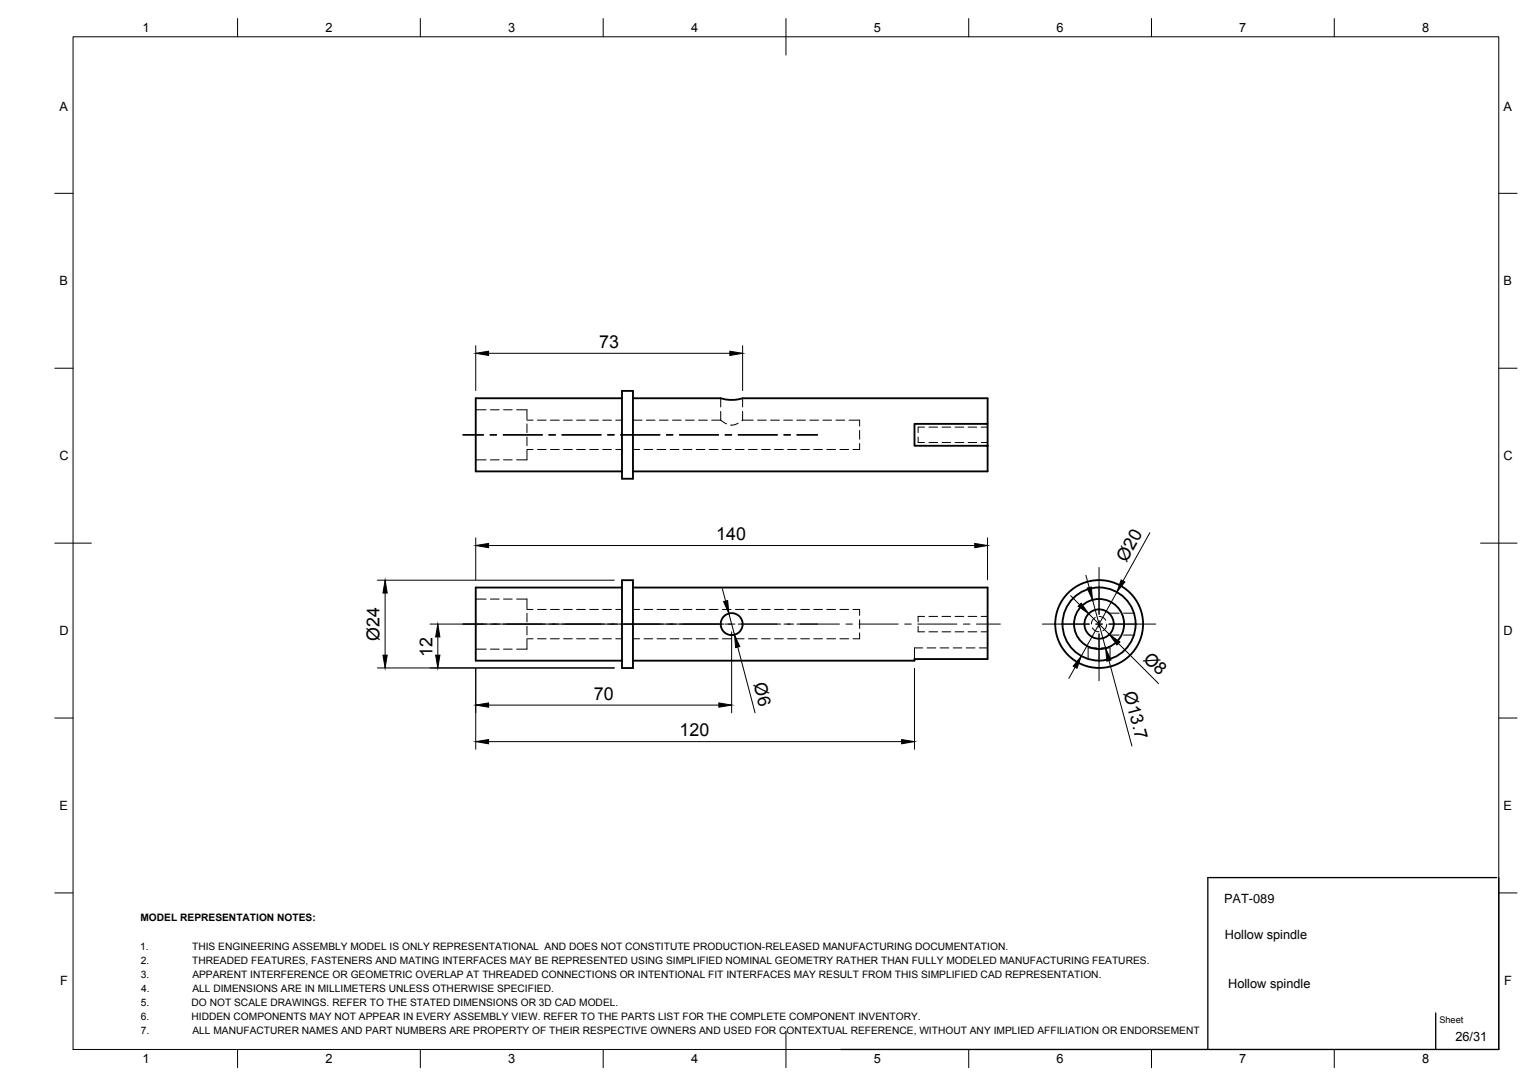
ISO-10303-21;
HEADER;
/* Generated by software containing ST-Developer
 * from STEP Tools, Inc. (www.steptools.com) 
 */

FILE_DESCRIPTION(
/* description */ ('Rotary union on bearing shaft'),
/* implementation_level */ '2;1');

FILE_NAME(
/* name */ 'Hollow spindle.step',
/* time_stamp */ '2026-10-28T03:24:01-07:00',
/* author */ (''),
/* organization */ (''),
/* preprocessor_version */ 'ST-DEVELOPER v20.2',
/* originating_system */ 'Autodesk Translation Framework v15.17.0.0',
/* authorisation */ '');

FILE_SCHEMA (('AUTOMOTIVE_DESIGN { 1 0 10303 214 3 1 1 }'));
ENDSEC;

DATA;
#10=MECHANICAL_DESIGN_GEOMETRIC_PRESENTATION_REPRESENTATION('',(#339),#9448);
#251=B_SPLINE_CURVE_WITH_KNOTS('',3,(#8795,#8796,#8797,#8798,#8799,#8800,
#8801,#8802,#8803,#8804,#8805,#8806,#8807,#8808,#8809,#8810,#8811,#8812),
 .UNSPECIFIED.,.F.,.F.,(4,2,2,2,2,2,2,2,4),(0.,0.113783176196775,0.22756635239355,
0.34131563198115,0.455064911568751,0.568814191156351,0.682563470743952,
0.796346646940726,0.910129823137501),.UNSPECIFIED.);
#252=B_SPLINE_CURVE_WITH_KNOTS('',3,(#8813,#8814,#8815,#8816,#8817,#8818,
#8819,#8820,#8821,#8822,#8823,#8824,#8825,#8826,#8827,#8828,#8829,#8830),
 .UNSPECIFIED.,.F.,.F.,(4,2,2,2,2,2,2,2,4),(0.910129823137501,1.02391299933428,
1.13769617553105,1.25144545511865,1.36519473470625,1.47894401429385,1.59269329388145,
1.70647647007823,1.820259646275),.UNSPECIFIED.);
#253=B_SPLINE_CURVE_WITH_KNOTS('',3,(#8865,#8866,#8867,#8868,#8869,#8870,
#8871,#8872,#8873,#8874,#8875,#8876,#8877,#8878,#8879,#8880,#8881,#8882,
#8883,#8884,#8885,#8886),.UNSPECIFIED.,.F.,.F.,(4,2,2,2,2,2,2,2,2,2,4),
(0.,0.0604340316452086,0.120868063290417,0.241736126580834,0.36006196705804,
0.478387807535245,0.596713648012451,0.715039488489656,0.835907551780074,
0.896341583425282,0.956775615070491),.UNSPECIFIED.);
#254=B_SPLINE_CURVE_WITH_KNOTS('',3,(#8887,#8888,#8889,#8890,#8891,#8892,
#8893,#8894,#8895,#8896,#8897,#8898,#8899,#8900,#8901,#8902,#8903,#8904,
#8905,#8906,#8907,#8908),.UNSPECIFIED.,.F.,.F.,(4,2,2,2,2,2,2,2,2,2,4),
(0.956775615070491,1.0172096467157,1.07764367836091,1.19851174165133,1.31683758212853,
1.43516342260574,1.55348926308294,1.67181510356015,1.79268316685056,1.85311719849577,
1.91355123014098),.UNSPECIFIED.);
#277=SHAPE_REPRESENTATION_RELATIONSHIP('SRR','None',#9579,#304);
#304=ADVANCED_BREP_SHAPE_REPRESENTATION('',(#372),#9439);
#339=STYLED_ITEM('',(#9764),#372);
#372=MANIFOLD_SOLID_BREP('Body1',#4896);
#455=FACE_BOUND('',#1233,.T.);
#456=FACE_BOUND('',#1235,.T.);
#457=FACE_BOUND('',#1238,.T.);
#458=FACE_BOUND('',#1245,.T.);
#459=FACE_BOUND('',#1248,.T.);
#460=FACE_BOUND('',#1251,.T.);
#461=FACE_BOUND('',#1253,.T.);
#589=PLANE('',#5618);
#590=PLANE('',#5619);
#591=PLANE('',#5620);
#592=PLANE('',#5622);
#593=PLANE('',#5623);
#594=PLANE('',#5628);
#595=PLANE('',#5630);
#596=PLANE('',#5632);
#597=PLANE('',#5635);
#598=PLANE('',#5645);
#599=PLANE('',#5649);
#600=PLANE('',#5650);
#601=PLANE('',#5651);
#852=FACE_OUTER_BOUND('',#1226,.T.);
#853=FACE_OUTER_BOUND('',#1227,.T.);
#854=FACE_OUTER_BOUND('',#1228,.T.);
#855=FACE_OUTER_BOUND('',#1229,.T.);
#856=FACE_OUTER_BOUND('',#1230,.T.);
#857=FACE_OUTER_BOUND('',#1231,.T.);
#858=FACE_OUTER_BOUND('',#1232,.T.);
#859=FACE_OUTER_BOUND('',#1234,.T.);
#860=FACE_OUTER_BOUND('',#1236,.T.);
#861=FACE_OUTER_BOUND('',#1237,.T.);
#862=FACE_OUTER_BOUND('',#1239,.T.);
#863=FACE_OUTER_BOUND('',#1240,.T.);
#864=FACE_OUTER_BOUND('',#1241,.T.);
#865=FACE_OUTER_BOUND('',#1242,.T.);
#866=FACE_OUTER_BOUND('',#1243,.T.);
#867=FACE_OUTER_BOUND('',#1244,.T.);
#868=FACE_OUTER_BOUND('',#1246,.T.);
#869=FACE_OUTER_BOUND('',#1247,.T.);
#870=FACE_OUTER_BOUND('',#1249,.T.);
#871=FACE_OUTER_BOUND('',#1250,.T.);
#872=FACE_OUTER_BOUND('',#1252,.T.);
#1226=EDGE_LOOP('',(#4063,#4064,#4065,#4066));
#1227=EDGE_LOOP('',(#4067));
#1228=EDGE_LOOP('',(#4068,#4069,#4070,#4071));
#1229=EDGE_LOOP('',(#4072,#4073,#4074,#4075));
#1230=EDGE_LOOP('',(#4076,#4077,#4078,#4079));
#1231=EDGE_LOOP('',(#4080,#4081,#4082,#4083));
#1232=EDGE_LOOP('',(#4084,#4085,#4086,#4087,#4088,#4089,#4090,#4091));
#1233=EDGE_LOOP('',(#4092,#4093));
#1234=EDGE_LOOP('',(#4094));
#1235=EDGE_LOOP('',(#4095));
#1236=EDGE_LOOP('',(#4096));
#1237=EDGE_LOOP('',(#4097));
#1238=EDGE_LOOP('',(#4098));
#1239=EDGE_LOOP('',(#4099));
#1240=EDGE_LOOP('',(#4100,#4101,#4102,#4103));
#1241=EDGE_LOOP('',(#4104,#4105,#4106,#4107));
#1242=EDGE_LOOP('',(#4108,#4109,#4110,#4111));
#1243=EDGE_LOOP('',(#4112,#4113,#4114,#4115));
#1244=EDGE_LOOP('',(#4116));
#1245=EDGE_LOOP('',(#4117));
#1246=EDGE_LOOP('',(#4118,#4119,#4120,#4121,#4122,#4123));
#1247=EDGE_LOOP('',(#4124,#4125,#4126,#4127));
#1248=EDGE_LOOP('',(#4128,#4129));
#1249=EDGE_LOOP('',(#4130));
#1250=EDGE_LOOP('',(#4131,#4132,#4133,#4134,#4135));
#1251=EDGE_LOOP('',(#4136));
#1252=EDGE_LOOP('',(#4137));
#1253=EDGE_LOOP('',(#4138));
#1546=LINE('',#8760,#1866);
#1547=LINE('',#8766,#1867);
#1548=LINE('',#8768,#1868);
#1549=LINE('',#8770,#1869);
#1550=LINE('',#8771,#1870);
#1551=LINE('',#8776,#1871);
#1552=LINE('',#8777,#1872);
#1553=LINE('',#8780,#1873);
#1554=LINE('',#8782,#1874);
#1555=LINE('',#8783,#1875);
#1556=LINE('',#8785,#1876);
#1557=LINE('',#8790,#1877);
#1558=LINE('',#8846,#1878);
#1559=LINE('',#8850,#1879);
#1560=LINE('',#8853,#1880);
#1561=LINE('',#8859,#1881);
#1562=LINE('',#8909,#1882);
#1563=LINE('',#8912,#1883);
#1866=VECTOR('',#6839,0.21);
#1867=VECTOR('',#6846,1.);
#1868=VECTOR('',#6847,1.);
#1869=VECTOR('',#6848,1.);
#1870=VECTOR('',#6849,1.);
#1871=VECTOR('',#6854,1.);
#1872=VECTOR('',#6855,1.);
#1873=VECTOR('',#6858,1.);
#1874=VECTOR('',#6859,1.);
#1875=VECTOR('',#6860,1.);
#1876=VECTOR('',#6863,1.);
#1877=VECTOR('',#6868,1.);
#1878=VECTOR('',#6893,1.2);
#1879=VECTOR('',#6898,0.4);
#1880=VECTOR('',#6901,1.);
#1881=VECTOR('',#6908,0.685);
#1882=VECTOR('',#6915,0.3);
#1883=VECTOR('',#6918,0.4);
#2188=CIRCLE('',#5616,0.21);
#2189=CIRCLE('',#5617,0.21);
#2190=CIRCLE('',#5621,1.);
#2191=CIRCLE('',#5625,1.);
#2192=CIRCLE('',#5626,1.);
#2193=CIRCLE('',#5627,1.);
#2194=CIRCLE('',#5629,1.2);
#2195=CIRCLE('',#5631,0.4);
#2196=CIRCLE('',#5633,1.2);
#2197=CIRCLE('',#5634,1.);
#2198=CIRCLE('',#5636,0.4);
#2199=CIRCLE('',#5639,0.4);
#2200=CIRCLE('',#5641,1.);
#2201=CIRCLE('',#5643,0.685);
#2202=CIRCLE('',#5644,0.685);
#2203=CIRCLE('',#5648,0.4);
#2524=VERTEX_POINT('',#8757);
#2525=VERTEX_POINT('',#8759);
#2526=VERTEX_POINT('',#8764);
#2527=VERTEX_POINT('',#8765);
#2528=VERTEX_POINT('',#8767);
#2529=VERTEX_POINT('',#8769);
#2530=VERTEX_POINT('',#8773);
#2531=VERTEX_POINT('',#8775);
#2532=VERTEX_POINT('',#8779);
#2533=VERTEX_POINT('',#8781);
#2534=VERTEX_POINT('',#8787);
#2535=VERTEX_POINT('',#8789);
#2536=VERTEX_POINT('',#8793);
#2537=VERTEX_POINT('',#8794);
#2538=VERTEX_POINT('',#8832);
#2539=VERTEX_POINT('',#8835);
#2540=VERTEX_POINT('',#8838);
#2541=VERTEX_POINT('',#8840);
#2542=VERTEX_POINT('',#8843);
#2543=VERTEX_POINT('',#8848);
#2544=VERTEX_POINT('',#8852);
#2545=VERTEX_POINT('',#8856);
#2546=VERTEX_POINT('',#8858);
#2547=VERTEX_POINT('',#8863);
#2548=VERTEX_POINT('',#8864);
#2549=VERTEX_POINT('',#8911);
#3059=EDGE_CURVE('',#2524,#2524,#2188,.T.);
#3060=EDGE_CURVE('',#2524,#2525,#1546,.T.);
#3061=EDGE_CURVE('',#2525,#2525,#2189,.T.);
#3062=EDGE_CURVE('',#2526,#2527,#1547,.T.);
#3063=EDGE_CURVE('',#2528,#2526,#1548,.T.);
#3064=EDGE_CURVE('',#2529,#2528,#1549,.T.);
#3065=EDGE_CURVE('',#2529,#2527,#1550,.T.);
#3066=EDGE_CURVE('',#2527,#2530,#2190,.T.);
#3067=EDGE_CURVE('',#2531,#2529,#1551,.T.);
#3068=EDGE_CURVE('',#2530,#2531,#1552,.T.);
#3069=EDGE_CURVE('',#2530,#2532,#1553,.T.);
#3070=EDGE_CURVE('',#2531,#2533,#1554,.T.);
#3071=EDGE_CURVE('',#2532,#2533,#1555,.T.);
#3072=EDGE_CURVE('',#2533,#2528,#1556,.T.);
#3073=EDGE_CURVE('',#2534,#2532,#2191,.T.);
#3074=EDGE_CURVE('',#2534,#2535,#1557,.T.);
#3075=EDGE_CURVE('',#2535,#2535,#2192,.T.);
#3076=EDGE_CURVE('',#2526,#2534,#2193,.T.);
#3077=EDGE_CURVE('',#2536,#2537,#251,.T.);
#3078=EDGE_CURVE('',#2537,#2536,#252,.T.);
#3079=EDGE_CURVE('',#2538,#2538,#2194,.T.);
#3080=EDGE_CURVE('',#2539,#2539,#2195,.T.);
#3081=EDGE_CURVE('',#2540,#2540,#2196,.T.);
#3082=EDGE_CURVE('',#2541,#2541,#2197,.T.);
#3083=EDGE_CURVE('',#2542,#2542,#2198,.T.);
#3084=EDGE_CURVE('',#2538,#2540,#1558,.T.);
#3085=EDGE_CURVE('',#2543,#2543,#2199,.T.);
#3086=EDGE_CURVE('',#2543,#2542,#1559,.T.);
#3087=EDGE_CURVE('',#2541,#2544,#1560,.T.);
#3088=EDGE_CURVE('',#2544,#2544,#2200,.T.);
#3089=EDGE_CURVE('',#2545,#2545,#2201,.T.);
#3090=EDGE_CURVE('',#2545,#2546,#1561,.T.);
#3091=EDGE_CURVE('',#2546,#2546,#2202,.T.);
#3092=EDGE_CURVE('',#2547,#2548,#253,.T.);
#3093=EDGE_CURVE('',#2548,#2547,#254,.T.);
#3094=EDGE_CURVE('',#2548,#2537,#1562,.T.);
#3095=EDGE_CURVE('',#2539,#2549,#1563,.T.);
#3096=EDGE_CURVE('',#2549,#2549,#2203,.T.);
#4063=ORIENTED_EDGE('',*,*,#3059,.F.);
#4064=ORIENTED_EDGE('',*,*,#3060,.T.);
#4065=ORIENTED_EDGE('',*,*,#3061,.F.);
#4066=ORIENTED_EDGE('',*,*,#3060,.F.);
#4067=ORIENTED_EDGE('',*,*,#3059,.T.);
#4068=ORIENTED_EDGE('',*,*,#3062,.F.);
#4069=ORIENTED_EDGE('',*,*,#3063,.F.);
#4070=ORIENTED_EDGE('',*,*,#3064,.F.);
#4071=ORIENTED_EDGE('',*,*,#3065,.T.);
#4072=ORIENTED_EDGE('',*,*,#3066,.F.);
#4073=ORIENTED_EDGE('',*,*,#3065,.F.);
#4074=ORIENTED_EDGE('',*,*,#3067,.F.);
#4075=ORIENTED_EDGE('',*,*,#3068,.F.);
#4076=ORIENTED_EDGE('',*,*,#3069,.F.);
#4077=ORIENTED_EDGE('',*,*,#3068,.T.);
#4078=ORIENTED_EDGE('',*,*,#3070,.T.);
#4079=ORIENTED_EDGE('',*,*,#3071,.F.);
#4080=ORIENTED_EDGE('',*,*,#3067,.T.);
#4081=ORIENTED_EDGE('',*,*,#3064,.T.);
#4082=ORIENTED_EDGE('',*,*,#3072,.F.);
#4083=ORIENTED_EDGE('',*,*,#3070,.F.);
#4084=ORIENTED_EDGE('',*,*,#3062,.T.);
#4085=ORIENTED_EDGE('',*,*,#3066,.T.);
#4086=ORIENTED_EDGE('',*,*,#3069,.T.);
#4087=ORIENTED_EDGE('',*,*,#3073,.F.);
#4088=ORIENTED_EDGE('',*,*,#3074,.T.);
#4089=ORIENTED_EDGE('',*,*,#3075,.T.);
#4090=ORIENTED_EDGE('',*,*,#3074,.F.);
#4091=ORIENTED_EDGE('',*,*,#3076,.F.);
#4092=ORIENTED_EDGE('',*,*,#3077,.T.);
#4093=ORIENTED_EDGE('',*,*,#3078,.T.);
#4094=ORIENTED_EDGE('',*,*,#3079,.T.);
#4095=ORIENTED_EDGE('',*,*,#3075,.F.);
#4096=ORIENTED_EDGE('',*,*,#3080,.F.);
#4097=ORIENTED_EDGE('',*,*,#3081,.F.);
#4098=ORIENTED_EDGE('',*,*,#3082,.F.);
#4099=ORIENTED_EDGE('',*,*,#3083,.F.);
#4100=ORIENTED_EDGE('',*,*,#3079,.F.);
#4101=ORIENTED_EDGE('',*,*,#3084,.T.);
#4102=ORIENTED_EDGE('',*,*,#3081,.T.);
#4103=ORIENTED_EDGE('',*,*,#3084,.F.);
#4104=ORIENTED_EDGE('',*,*,#3085,.T.);
#4105=ORIENTED_EDGE('',*,*,#3086,.T.);
#4106=ORIENTED_EDGE('',*,*,#3083,.T.);
#4107=ORIENTED_EDGE('',*,*,#3086,.F.);
#4108=ORIENTED_EDGE('',*,*,#3082,.T.);
#4109=ORIENTED_EDGE('',*,*,#3087,.T.);
#4110=ORIENTED_EDGE('',*,*,#3088,.T.);
#4111=ORIENTED_EDGE('',*,*,#3087,.F.);
#4112=ORIENTED_EDGE('',*,*,#3089,.F.);
#4113=ORIENTED_EDGE('',*,*,#3090,.T.);
#4114=ORIENTED_EDGE('',*,*,#3091,.T.);
#4115=ORIENTED_EDGE('',*,*,#3090,.F.);
#4116=ORIENTED_EDGE('',*,*,#3091,.F.);
#4117=ORIENTED_EDGE('',*,*,#3085,.F.);
#4118=ORIENTED_EDGE('',*,*,#3092,.F.);
#4119=ORIENTED_EDGE('',*,*,#3093,.F.);
#4120=ORIENTED_EDGE('',*,*,#3094,.T.);
#4121=ORIENTED_EDGE('',*,*,#3077,.F.);
#4122=ORIENTED_EDGE('',*,*,#3078,.F.);
#4123=ORIENTED_EDGE('',*,*,#3094,.F.);
#4124=ORIENTED_EDGE('',*,*,#3080,.T.);
#4125=ORIENTED_EDGE('',*,*,#3095,.T.);
#4126=ORIENTED_EDGE('',*,*,#3096,.T.);
#4127=ORIENTED_EDGE('',*,*,#3095,.F.);
#4128=ORIENTED_EDGE('',*,*,#3092,.T.);
#4129=ORIENTED_EDGE('',*,*,#3093,.T.);
#4130=ORIENTED_EDGE('',*,*,#3096,.F.);
#4131=ORIENTED_EDGE('',*,*,#3063,.T.);
#4132=ORIENTED_EDGE('',*,*,#3076,.T.);
#4133=ORIENTED_EDGE('',*,*,#3073,.T.);
#4134=ORIENTED_EDGE('',*,*,#3071,.T.);
#4135=ORIENTED_EDGE('',*,*,#3072,.T.);
#4136=ORIENTED_EDGE('',*,*,#3061,.T.);
#4137=ORIENTED_EDGE('',*,*,#3088,.F.);
#4138=ORIENTED_EDGE('',*,*,#3089,.T.);
#4541=CYLINDRICAL_SURFACE('',#5615,0.21);
#4542=CYLINDRICAL_SURFACE('',#5624,1.);
#4543=CYLINDRICAL_SURFACE('',#5637,1.2);
#4544=CYLINDRICAL_SURFACE('',#5638,0.4);
#4545=CYLINDRICAL_SURFACE('',#5640,1.);
#4546=CYLINDRICAL_SURFACE('',#5642,0.685);
#4547=CYLINDRICAL_SURFACE('',#5646,0.3);
#4548=CYLINDRICAL_SURFACE('',#5647,0.4);
#4765=ADVANCED_FACE('',(#852),#4541,.F.);
#4766=ADVANCED_FACE('',(#853),#589,.T.);
#4767=ADVANCED_FACE('',(#854),#590,.F.);
#4768=ADVANCED_FACE('',(#855),#591,.T.);
#4769=ADVANCED_FACE('',(#856),#592,.F.);
#4770=ADVANCED_FACE('',(#857),#593,.F.);
#4771=ADVANCED_FACE('',(#858,#455),#4542,.T.);
#4772=ADVANCED_FACE('',(#859,#456),#594,.T.);
#4773=ADVANCED_FACE('',(#860),#595,.T.);
#4774=ADVANCED_FACE('',(#861,#457),#596,.F.);
#4775=ADVANCED_FACE('',(#862),#597,.F.);
#4776=ADVANCED_FACE('',(#863),#4543,.T.);
#4777=ADVANCED_FACE('',(#864),#4544,.F.);
#4778=ADVANCED_FACE('',(#865),#4545,.T.);
#4779=ADVANCED_FACE('',(#866),#4546,.F.);
#4780=ADVANCED_FACE('',(#867,#458),#598,.F.);
#4781=ADVANCED_FACE('',(#868),#4547,.F.);
#4782=ADVANCED_FACE('',(#869,#459),#4548,.F.);
#4783=ADVANCED_FACE('',(#870),#599,.F.);
#4784=ADVANCED_FACE('',(#871,#460),#600,.T.);
#4785=ADVANCED_FACE('',(#872,#461),#601,.F.);
#4896=CLOSED_SHELL('',(#4765,#4766,#4767,#4768,#4769,#4770,#4771,#4772,
#4773,#4774,#4775,#4776,#4777,#4778,#4779,#4780,#4781,#4782,#4783,#4784,
#4785));
#5614=AXIS2_PLACEMENT_3D('',#8755,#6833,#6834);
#5615=AXIS2_PLACEMENT_3D('',#8756,#6835,#6836);
#5616=AXIS2_PLACEMENT_3D('',#8758,#6837,#6838);
#5617=AXIS2_PLACEMENT_3D('',#8761,#6840,#6841);
#5618=AXIS2_PLACEMENT_3D('',#8762,#6842,#6843);
#5619=AXIS2_PLACEMENT_3D('',#8763,#6844,#6845);
#5620=AXIS2_PLACEMENT_3D('',#8772,#6850,#6851);
#5621=AXIS2_PLACEMENT_3D('',#8774,#6852,#6853);
#5622=AXIS2_PLACEMENT_3D('',#8778,#6856,#6857);
#5623=AXIS2_PLACEMENT_3D('',#8784,#6861,#6862);
#5624=AXIS2_PLACEMENT_3D('',#8786,#6864,#6865);
#5625=AXIS2_PLACEMENT_3D('',#8788,#6866,#6867);
#5626=AXIS2_PLACEMENT_3D('',#8791,#6869,#6870);
#5627=AXIS2_PLACEMENT_3D('',#8792,#6871,#6872);
#5628=AXIS2_PLACEMENT_3D('',#8831,#6873,#6874);
#5629=AXIS2_PLACEMENT_3D('',#8833,#6875,#6876);
#5630=AXIS2_PLACEMENT_3D('',#8834,#6877,#6878);
#5631=AXIS2_PLACEMENT_3D('',#8836,#6879,#6880);
#5632=AXIS2_PLACEMENT_3D('',#8837,#6881,#6882);
#5633=AXIS2_PLACEMENT_3D('',#8839,#6883,#6884);
#5634=AXIS2_PLACEMENT_3D('',#8841,#6885,#6886);
#5635=AXIS2_PLACEMENT_3D('',#8842,#6887,#6888);
#5636=AXIS2_PLACEMENT_3D('',#8844,#6889,#6890);
#5637=AXIS2_PLACEMENT_3D('',#8845,#6891,#6892);
#5638=AXIS2_PLACEMENT_3D('',#8847,#6894,#6895);
#5639=AXIS2_PLACEMENT_3D('',#8849,#6896,#6897);
#5640=AXIS2_PLACEMENT_3D('',#8851,#6899,#6900);
#5641=AXIS2_PLACEMENT_3D('',#8854,#6902,#6903);
#5642=AXIS2_PLACEMENT_3D('',#8855,#6904,#6905);
#5643=AXIS2_PLACEMENT_3D('',#8857,#6906,#6907);
#5644=AXIS2_PLACEMENT_3D('',#8860,#6909,#6910);
#5645=AXIS2_PLACEMENT_3D('',#8861,#6911,#6912);
#5646=AXIS2_PLACEMENT_3D('',#8862,#6913,#6914);
#5647=AXIS2_PLACEMENT_3D('',#8910,#6916,#6917);
#5648=AXIS2_PLACEMENT_3D('',#8913,#6919,#6920);
#5649=AXIS2_PLACEMENT_3D('',#8914,#6921,#6922);
#5650=AXIS2_PLACEMENT_3D('',#8915,#6923,#6924);
#5651=AXIS2_PLACEMENT_3D('',#8916,#6925,#6926);
#6833=DIRECTION('axis',(0.,0.,1.));
#6834=DIRECTION('refdir',(1.,0.,0.));
#6835=DIRECTION('center_axis',(0.,1.,0.));
#6836=DIRECTION('ref_axis',(1.,0.,0.));
#6837=DIRECTION('center_axis',(0.,1.,0.));
#6838=DIRECTION('ref_axis',(1.,0.,0.));
#6839=DIRECTION('',(0.,1.,0.));
#6840=DIRECTION('center_axis',(0.,-1.,0.));
#6841=DIRECTION('ref_axis',(1.,0.,0.));
#6842=DIRECTION('center_axis',(0.,1.,0.));
#6843=DIRECTION('ref_axis',(1.,0.,0.));
#6844=DIRECTION('center_axis',(-1.,0.,0.));
#6845=DIRECTION('ref_axis',(0.,0.,1.));
#6846=DIRECTION('',(0.,-1.,0.));
#6847=DIRECTION('',(0.,0.,-1.));
#6848=DIRECTION('',(0.,1.,0.));
#6849=DIRECTION('',(0.,0.,-1.));
#6850=DIRECTION('center_axis',(0.,1.,0.));
#6851=DIRECTION('ref_axis',(1.,0.,0.));
#6852=DIRECTION('center_axis',(0.,-1.,0.));
#6853=DIRECTION('ref_axis',(1.,0.,0.));
#6854=DIRECTION('',(-1.,0.,0.));
#6855=DIRECTION('',(0.,0.,1.));
#6856=DIRECTION('center_axis',(1.,0.,0.));
#6857=DIRECTION('ref_axis',(0.,0.,-1.));
#6858=DIRECTION('',(0.,1.,0.));
#6859=DIRECTION('',(0.,1.,0.));
#6860=DIRECTION('',(0.,0.,1.));
#6861=DIRECTION('center_axis',(0.,0.,1.));
#6862=DIRECTION('ref_axis',(1.,0.,0.));
#6863=DIRECTION('',(-1.,0.,0.));
#6864=DIRECTION('center_axis',(0.,1.,0.));
#6865=DIRECTION('ref_axis',(1.,0.,0.));
#6866=DIRECTION('center_axis',(0.,1.,0.));
#6867=DIRECTION('ref_axis',(1.,0.,0.));
#6868=DIRECTION('',(0.,-1.,0.));
#6869=DIRECTION('center_axis',(0.,1.,0.));
#6870=DIRECTION('ref_axis',(1.,0.,0.));
#6871=DIRECTION('center_axis',(0.,1.,0.));
#6872=DIRECTION('ref_axis',(1.,0.,0.));
#6873=DIRECTION('center_axis',(0.,1.,0.));
#6874=DIRECTION('ref_axis',(1.,0.,0.));
#6875=DIRECTION('center_axis',(0.,1.,0.));
#6876=DIRECTION('ref_axis',(1.,0.,0.));
#6877=DIRECTION('center_axis',(0.,1.,0.));
#6878=DIRECTION('ref_axis',(1.,0.,0.));
#6879=DIRECTION('center_axis',(0.,-1.,0.));
#6880=DIRECTION('ref_axis',(1.,0.,0.));
#6881=DIRECTION('center_axis',(0.,1.,0.));
#6882=DIRECTION('ref_axis',(1.,0.,0.));
#6883=DIRECTION('center_axis',(0.,1.,0.));
#6884=DIRECTION('ref_axis',(1.,0.,0.));
#6885=DIRECTION('center_axis',(0.,-1.,0.));
#6886=DIRECTION('ref_axis',(1.,0.,0.));
#6887=DIRECTION('center_axis',(0.,1.,0.));
#6888=DIRECTION('ref_axis',(1.,0.,0.));
#6889=DIRECTION('center_axis',(0.,1.,0.));
#6890=DIRECTION('ref_axis',(1.,0.,0.));
#6891=DIRECTION('center_axis',(0.,1.,0.));
#6892=DIRECTION('ref_axis',(1.,0.,0.));
#6893=DIRECTION('',(0.,-1.,0.));
#6894=DIRECTION('center_axis',(0.,1.,0.));
#6895=DIRECTION('ref_axis',(1.,0.,0.));
#6896=DIRECTION('center_axis',(0.,-1.,0.));
#6897=DIRECTION('ref_axis',(1.,0.,0.));
#6898=DIRECTION('',(0.,1.,0.));
#6899=DIRECTION('center_axis',(0.,1.,0.));
#6900=DIRECTION('ref_axis',(1.,0.,0.));
#6901=DIRECTION('',(0.,-1.,0.));
#6902=DIRECTION('center_axis',(0.,1.,0.));
#6903=DIRECTION('ref_axis',(1.,0.,0.));
#6904=DIRECTION('center_axis',(0.,1.,0.));
#6905=DIRECTION('ref_axis',(1.,0.,0.));
#6906=DIRECTION('center_axis',(0.,1.,0.));
#6907=DIRECTION('ref_axis',(1.,0.,0.));
#6908=DIRECTION('',(0.,1.,0.));
#6909=DIRECTION('center_axis',(0.,1.,0.));
#6910=DIRECTION('ref_axis',(1.,0.,0.));
#6911=DIRECTION('center_axis',(0.,1.,0.));
#6912=DIRECTION('ref_axis',(1.,0.,0.));
#6913=DIRECTION('center_axis',(1.,0.,0.));
#6914=DIRECTION('ref_axis',(0.,0.,-1.));
#6915=DIRECTION('',(1.,0.,0.));
#6916=DIRECTION('center_axis',(0.,1.,0.));
#6917=DIRECTION('ref_axis',(1.,0.,0.));
#6918=DIRECTION('',(0.,1.,0.));
#6919=DIRECTION('center_axis',(0.,1.,0.));
#6920=DIRECTION('ref_axis',(1.,0.,0.));
#6921=DIRECTION('center_axis',(0.,1.,0.));
#6922=DIRECTION('ref_axis',(1.,0.,0.));
#6923=DIRECTION('center_axis',(0.,1.,0.));
#6924=DIRECTION('ref_axis',(1.,0.,0.));
#6925=DIRECTION('center_axis',(0.,1.,0.));
#6926=DIRECTION('ref_axis',(1.,0.,0.));
#8755=CARTESIAN_POINT('',(0.,0.,0.));
#8756=CARTESIAN_POINT('Origin',(0.,8.1,4.5));
#8757=CARTESIAN_POINT('',(-0.21,8.1,4.5));
#8758=CARTESIAN_POINT('Origin',(0.,8.1,4.5));
#8759=CARTESIAN_POINT('',(-0.21,10.,4.5));
#8760=CARTESIAN_POINT('',(-0.21,8.1,4.5));
#8761=CARTESIAN_POINT('Origin',(0.,10.,4.5));
#8762=CARTESIAN_POINT('Origin',(0.,8.1,4.5));
#8763=CARTESIAN_POINT('Origin',(-0.3,8.,3.4));
#8764=CARTESIAN_POINT('',(-0.3,10.,3.54606079858305));
#8765=CARTESIAN_POINT('',(-0.3,8.,3.54606079858305));
#8766=CARTESIAN_POINT('',(-0.3,-4.,3.54606079858305));
#8767=CARTESIAN_POINT('',(-0.3,10.,3.85));
#8768=CARTESIAN_POINT('',(-0.3,10.,3.95));
#8769=CARTESIAN_POINT('',(-0.3,8.,3.85));
#8770=CARTESIAN_POINT('',(-0.3,8.,3.85));
#8771=CARTESIAN_POINT('',(-0.3,8.,3.85));
#8772=CARTESIAN_POINT('Origin',(0.,8.,3.625));
#8773=CARTESIAN_POINT('',(0.3,8.,3.54606079858305));
#8774=CARTESIAN_POINT('Origin',(0.,8.,4.5));
#8775=CARTESIAN_POINT('',(0.3,8.,3.85));
#8776=CARTESIAN_POINT('',(0.3,8.,3.85));
#8777=CARTESIAN_POINT('',(0.3,8.,3.4));
#8778=CARTESIAN_POINT('Origin',(0.3,8.,3.85));
#8779=CARTESIAN_POINT('',(0.3,10.,3.54606079858305));
#8780=CARTESIAN_POINT('',(0.3,-4.,3.54606079858305));
#8781=CARTESIAN_POINT('',(0.3,10.,3.85));
#8782=CARTESIAN_POINT('',(0.3,8.,3.85));
#8783=CARTESIAN_POINT('',(0.3,10.,4.175));
#8784=CARTESIAN_POINT('Origin',(-0.3,8.,3.85));
#8785=CARTESIAN_POINT('',(-0.15,10.,3.85));
#8786=CARTESIAN_POINT('Origin',(0.,-4.,4.5));
#8787=CARTESIAN_POINT('',(-1.,10.,4.5));
#8788=CARTESIAN_POINT('Origin',(0.,10.,4.5));
#8789=CARTESIAN_POINT('',(-1.,0.3,4.5));
#8790=CARTESIAN_POINT('',(-1.,-4.,4.5));
#8791=CARTESIAN_POINT('Origin',(0.,0.3,4.5));
#8792=CARTESIAN_POINT('Origin',(0.,10.,4.5));
#8793=CARTESIAN_POINT('',(0.953939201416946,3.,4.2));
#8794=CARTESIAN_POINT('',(0.953939201416946,3.,4.8));
#8795=CARTESIAN_POINT('Ctrl Pts',(0.953939201416946,3.,4.2));
#8796=CARTESIAN_POINT('Ctrl Pts',(0.953939201416946,2.96207227460108,4.2));
#8797=CARTESIAN_POINT('Ctrl Pts',(0.956437939057488,2.92178925145718,4.20762790839008));
#8798=CARTESIAN_POINT('Ctrl Pts',(0.965284956103208,2.84795244622839,4.23831332738424));
#8799=CARTESIAN_POINT('Ctrl Pts',(0.971486751729016,2.81437646254953,4.26135946873854));
#8800=CARTESIAN_POINT('Ctrl Pts',(0.982993562614982,2.76136736575978,4.31436856552829));
#8801=CARTESIAN_POINT('Ctrl Pts',(0.98907119499008,2.7383151092967,4.34794775809938));
#8802=CARTESIAN_POINT('Ctrl Pts',(0.997630133387832,2.70762517534893,4.42179622825181));
#8803=CARTESIAN_POINT('Ctrl Pts',(1.,2.7,4.4620835734708));
#8804=CARTESIAN_POINT('Ctrl Pts',(1.,2.7,4.5379164265292));
#8805=CARTESIAN_POINT('Ctrl Pts',(0.997630133387832,2.70762517534893,4.57820377174819));
#8806=CARTESIAN_POINT('Ctrl Pts',(0.98907119499008,2.7383151092967,4.65205224190062));
#8807=CARTESIAN_POINT('Ctrl Pts',(0.982993562614982,2.76136736575978,4.68563143447171));
#8808=CARTESIAN_POINT('Ctrl Pts',(0.971486751729016,2.81437646254953,4.73864053126146));
#8809=CARTESIAN_POINT('Ctrl Pts',(0.965284956103208,2.84795244622839,4.76168667261576));
#8810=CARTESIAN_POINT('Ctrl Pts',(0.956437939057488,2.92178925145718,4.79237209160992));
#8811=CARTESIAN_POINT('Ctrl Pts',(0.953939201416946,2.96207227460107,4.8));
#8812=CARTESIAN_POINT('Ctrl Pts',(0.953939201416946,3.,4.8));
#8813=CARTESIAN_POINT('Ctrl Pts',(0.953939201416946,3.,4.8));
#8814=CARTESIAN_POINT('Ctrl Pts',(0.953939201416946,3.03792772539892,4.8));
#8815=CARTESIAN_POINT('Ctrl Pts',(0.956437939057488,3.07821074854282,4.79237209160992));
#8816=CARTESIAN_POINT('Ctrl Pts',(0.965284956103208,3.15204755377161,4.76168667261577));
#8817=CARTESIAN_POINT('Ctrl Pts',(0.971486751729016,3.18562353745047,4.73864053126146));
#8818=CARTESIAN_POINT('Ctrl Pts',(0.982993562614982,3.23863263424022,4.68563143447171));
#8819=CARTESIAN_POINT('Ctrl Pts',(0.98907119499008,3.2616848907033,4.65205224190062));
#8820=CARTESIAN_POINT('Ctrl Pts',(0.997630133387832,3.29237482465107,4.57820377174819));
#8821=CARTESIAN_POINT('Ctrl Pts',(1.,3.3,4.5379164265292));
#8822=CARTESIAN_POINT('Ctrl Pts',(1.,3.3,4.4620835734708));
#8823=CARTESIAN_POINT('Ctrl Pts',(0.997630133387832,3.29237482465107,4.42179622825181));
#8824=CARTESIAN_POINT('Ctrl Pts',(0.98907119499008,3.2616848907033,4.34794775809938));
#8825=CARTESIAN_POINT('Ctrl Pts',(0.982993562614982,3.23863263424022,4.31436856552829));
#8826=CARTESIAN_POINT('Ctrl Pts',(0.971486751729016,3.18562353745047,4.26135946873854));
#8827=CARTESIAN_POINT('Ctrl Pts',(0.965284956103208,3.15204755377161,4.23831332738423));
#8828=CARTESIAN_POINT('Ctrl Pts',(0.956437939057488,3.07821074854282,4.20762790839008));
#8829=CARTESIAN_POINT('Ctrl Pts',(0.953939201416946,3.03792772539892,4.2));
#8830=CARTESIAN_POINT('Ctrl Pts',(0.953939201416946,3.,4.2));
#8831=CARTESIAN_POINT('Origin',(0.,0.3,4.5));
#8832=CARTESIAN_POINT('',(-1.2,0.3,4.5));
#8833=CARTESIAN_POINT('Origin',(0.,0.3,4.5));
#8834=CARTESIAN_POINT('Origin',(0.,0.3,4.5));
#8835=CARTESIAN_POINT('',(-0.4,0.3,4.5));
#8836=CARTESIAN_POINT('Origin',(0.,0.3,4.5));
#8837=CARTESIAN_POINT('Origin',(0.,0.,4.5));
#8838=CARTESIAN_POINT('',(-1.2,0.,4.5));
#8839=CARTESIAN_POINT('Origin',(0.,0.,4.5));
#8840=CARTESIAN_POINT('',(-1.,0.,4.5));
#8841=CARTESIAN_POINT('Origin',(0.,0.,4.5));
#8842=CARTESIAN_POINT('Origin',(0.,0.,4.5));
#8843=CARTESIAN_POINT('',(-0.4,0.,4.5));
#8844=CARTESIAN_POINT('Origin',(0.,0.,4.5));
#8845=CARTESIAN_POINT('Origin',(0.,0.,4.5));
#8846=CARTESIAN_POINT('',(-1.2,0.,4.5));
#8847=CARTESIAN_POINT('Origin',(0.,-4.1,4.5));
#8848=CARTESIAN_POINT('',(-0.4,-2.6,4.5));
#8849=CARTESIAN_POINT('Origin',(0.,-2.6,4.5));
#8850=CARTESIAN_POINT('',(-0.4,-4.1,4.5));
#8851=CARTESIAN_POINT('Origin',(0.,-4.,4.5));
#8852=CARTESIAN_POINT('',(-1.,-4.,4.5));
#8853=CARTESIAN_POINT('',(-1.,-4.,4.5));
#8854=CARTESIAN_POINT('Origin',(0.,-4.,4.5));
#8855=CARTESIAN_POINT('Origin',(0.,-4.1,4.5));
#8856=CARTESIAN_POINT('',(-0.685,-4.,4.5));
#8857=CARTESIAN_POINT('Origin',(0.,-4.,4.5));
#8858=CARTESIAN_POINT('',(-0.685,-2.6,4.5));
#8859=CARTESIAN_POINT('',(-0.685,-4.1,4.5));
#8860=CARTESIAN_POINT('Origin',(0.,-2.6,4.5));
#8861=CARTESIAN_POINT('Origin',(0.,-2.6,4.5));
#8862=CARTESIAN_POINT('Origin',(0.,3.,4.5));
#8863=CARTESIAN_POINT('',(0.264575131106459,3.,4.2));
#8864=CARTESIAN_POINT('',(0.264575131106459,3.,4.8));
#8865=CARTESIAN_POINT('Ctrl Pts',(0.264575131106459,3.,4.2));
#8866=CARTESIAN_POINT('Ctrl Pts',(0.264575131106459,3.02014467721507,4.2));
#8867=CARTESIAN_POINT('Ctrl Pts',(0.266946656583194,3.0403635841556,4.2020492278835));
#8868=CARTESIAN_POINT('Ctrl Pts',(0.275663470560297,3.07974365991683,4.21009513514317));
#8869=CARTESIAN_POINT('Ctrl Pts',(0.281970270384709,3.09891429794725,4.21608711674642));
#8870=CARTESIAN_POINT('Ctrl Pts',(0.304063569802551,3.15349908017058,4.2392312552828));
#8871=CARTESIAN_POINT('Ctrl Pts',(0.322818652826944,3.18607812595988,4.26181405724795));
#8872=CARTESIAN_POINT('Ctrl Pts',(0.35507155223138,3.23763794985389,4.31337388114196));
#8873=CARTESIAN_POINT('Ctrl Pts',(0.371172434841458,3.26054860088286,4.34601764444721));
#8874=CARTESIAN_POINT('Ctrl Pts',(0.393713960479867,3.29176580029427,4.41957074694018));
#8875=CARTESIAN_POINT('Ctrl Pts',(0.4,3.3,4.46055805317426));
#8876=CARTESIAN_POINT('Ctrl Pts',(0.4,3.3,4.53944194682574));
#8877=CARTESIAN_POINT('Ctrl Pts',(0.393713960479867,3.29176580029427,4.58042925305982));
#8878=CARTESIAN_POINT('Ctrl Pts',(0.371172434841458,3.26054860088286,4.65398235555279));
#8879=CARTESIAN_POINT('Ctrl Pts',(0.35507155223138,3.23763794985389,4.68662611885804));
#8880=CARTESIAN_POINT('Ctrl Pts',(0.322818652826944,3.18607812595988,4.73818594275205));
#8881=CARTESIAN_POINT('Ctrl Pts',(0.304063569802551,3.15349908017058,4.7607687447172));
#8882=CARTESIAN_POINT('Ctrl Pts',(0.281970270384709,3.09891429794725,4.78391288325358));
#8883=CARTESIAN_POINT('Ctrl Pts',(0.275663470560297,3.07974365991683,4.78990486485683));
#8884=CARTESIAN_POINT('Ctrl Pts',(0.266946656583194,3.0403635841556,4.7979507721165));
#8885=CARTESIAN_POINT('Ctrl Pts',(0.264575131106459,3.02014467721507,4.8));
#8886=CARTESIAN_POINT('Ctrl Pts',(0.264575131106459,3.,4.8));
#8887=CARTESIAN_POINT('Ctrl Pts',(0.264575131106459,3.,4.8));
#8888=CARTESIAN_POINT('Ctrl Pts',(0.264575131106459,2.97985532278493,4.8));
#8889=CARTESIAN_POINT('Ctrl Pts',(0.266946656583194,2.9596364158444,4.7979507721165));
#8890=CARTESIAN_POINT('Ctrl Pts',(0.275663470560297,2.92025634008317,4.78990486485683));
#8891=CARTESIAN_POINT('Ctrl Pts',(0.281970270384709,2.90108570205275,4.78391288325358));
#8892=CARTESIAN_POINT('Ctrl Pts',(0.304063569802551,2.84650091982942,4.7607687447172));
#8893=CARTESIAN_POINT('Ctrl Pts',(0.322818652826944,2.81392187404012,4.73818594275205));
#8894=CARTESIAN_POINT('Ctrl Pts',(0.35507155223138,2.76236205014611,4.68662611885804));
#8895=CARTESIAN_POINT('Ctrl Pts',(0.371172434841458,2.73945139911714,4.65398235555279));
#8896=CARTESIAN_POINT('Ctrl Pts',(0.393713960479867,2.70823419970573,4.58042925305983));
#8897=CARTESIAN_POINT('Ctrl Pts',(0.4,2.7,4.53944194682573));
#8898=CARTESIAN_POINT('Ctrl Pts',(0.4,2.7,4.46055805317426));
#8899=CARTESIAN_POINT('Ctrl Pts',(0.393713960479867,2.70823419970573,4.41957074694017));
#8900=CARTESIAN_POINT('Ctrl Pts',(0.371172434841458,2.73945139911714,4.34601764444721));
#8901=CARTESIAN_POINT('Ctrl Pts',(0.35507155223138,2.76236205014611,4.31337388114196));
#8902=CARTESIAN_POINT('Ctrl Pts',(0.322818652826944,2.81392187404012,4.26181405724795));
#8903=CARTESIAN_POINT('Ctrl Pts',(0.304063569802551,2.84650091982942,4.2392312552828));
#8904=CARTESIAN_POINT('Ctrl Pts',(0.281970270384709,2.90108570205275,4.21608711674642));
#8905=CARTESIAN_POINT('Ctrl Pts',(0.275663470560297,2.92025634008317,4.21009513514317));
#8906=CARTESIAN_POINT('Ctrl Pts',(0.266946656583194,2.9596364158444,4.2020492278835));
#8907=CARTESIAN_POINT('Ctrl Pts',(0.264575131106459,2.97985532278493,4.2));
#8908=CARTESIAN_POINT('Ctrl Pts',(0.264575131106459,3.,4.2));
#8909=CARTESIAN_POINT('',(0.,3.,4.8));
#8910=CARTESIAN_POINT('Origin',(0.,-4.1,4.5));
#8911=CARTESIAN_POINT('',(-0.4,6.5,4.5));
#8912=CARTESIAN_POINT('',(-0.4,-4.1,4.5));
#8913=CARTESIAN_POINT('Origin',(0.,6.5,4.5));
#8914=CARTESIAN_POINT('Origin',(0.,6.5,4.5));
#8915=CARTESIAN_POINT('Origin',(0.,10.,4.5));
#8916=CARTESIAN_POINT('Origin',(0.,-4.,4.5));
#9407=UNCERTAINTY_MEASURE_WITH_UNIT(LENGTH_MEASURE(0.001),#9449,
'DISTANCE_ACCURACY_VALUE',
'Maximum model space distance between geometric entities at asserted c
onnectivities');
#9416=UNCERTAINTY_MEASURE_WITH_UNIT(LENGTH_MEASURE(0.001),#9449,
'DISTANCE_ACCURACY_VALUE',
'Maximum model space distance between geometric entities at asserted c
onnectivities');
#9439=(
GEOMETRIC_REPRESENTATION_CONTEXT(3)
GLOBAL_UNCERTAINTY_ASSIGNED_CONTEXT((#9407))
GLOBAL_UNIT_ASSIGNED_CONTEXT((#9449,#9451,#9452))
REPRESENTATION_CONTEXT('','3D')
);
#9448=(
GEOMETRIC_REPRESENTATION_CONTEXT(3)
GLOBAL_UNCERTAINTY_ASSIGNED_CONTEXT((#9416))
GLOBAL_UNIT_ASSIGNED_CONTEXT((#9449,#9451,#9452))
REPRESENTATION_CONTEXT('','3D')
);
#9449=(
LENGTH_UNIT()
NAMED_UNIT(*)
SI_UNIT(.CENTI.,.METRE.)
);
#9451=(
NAMED_UNIT(*)
PLANE_ANGLE_UNIT()
SI_UNIT($,.RADIAN.)
);
#9452=(
NAMED_UNIT(*)
SI_UNIT($,.STERADIAN.)
SOLID_ANGLE_UNIT()
);
#9475=SHAPE_DEFINITION_REPRESENTATION(#9511,#9579);
#9511=PRODUCT_DEFINITION_SHAPE('',$,#9611);
#9579=SHAPE_REPRESENTATION('',(#5614),#9439);
#9588=PRODUCT_DEFINITION_CONTEXT('part definition',#9683,'design');
#9611=PRODUCT_DEFINITION('Hollow spindle','Hollow spindle',#9642,#9588);
#9642=PRODUCT_DEFINITION_FORMATION('',$,#9707);
#9683=APPLICATION_CONTEXT(
'Core Data for Automotive Mechanical Design Process');
#9684=PRODUCT_CONTEXT('part definition',#9683,'mechanical');
#9707=PRODUCT('Hollow spindle','Hollow spindle','Hollow spindle',(#9684));
#9758=COLOUR_RGB('Light Blue',0.38,0.62,0.78);
#9759=FILL_AREA_STYLE_COLOUR('',#9758);
#9760=FILL_AREA_STYLE('',(#9759));
#9761=SURFACE_STYLE_FILL_AREA(#9760);
#9762=SURFACE_SIDE_STYLE('',(#9761));
#9763=SURFACE_STYLE_USAGE(.BOTH.,#9762);
#9764=PRESENTATION_STYLE_ASSIGNMENT((#9763));
ENDSEC;
END-ISO-10303-21;
